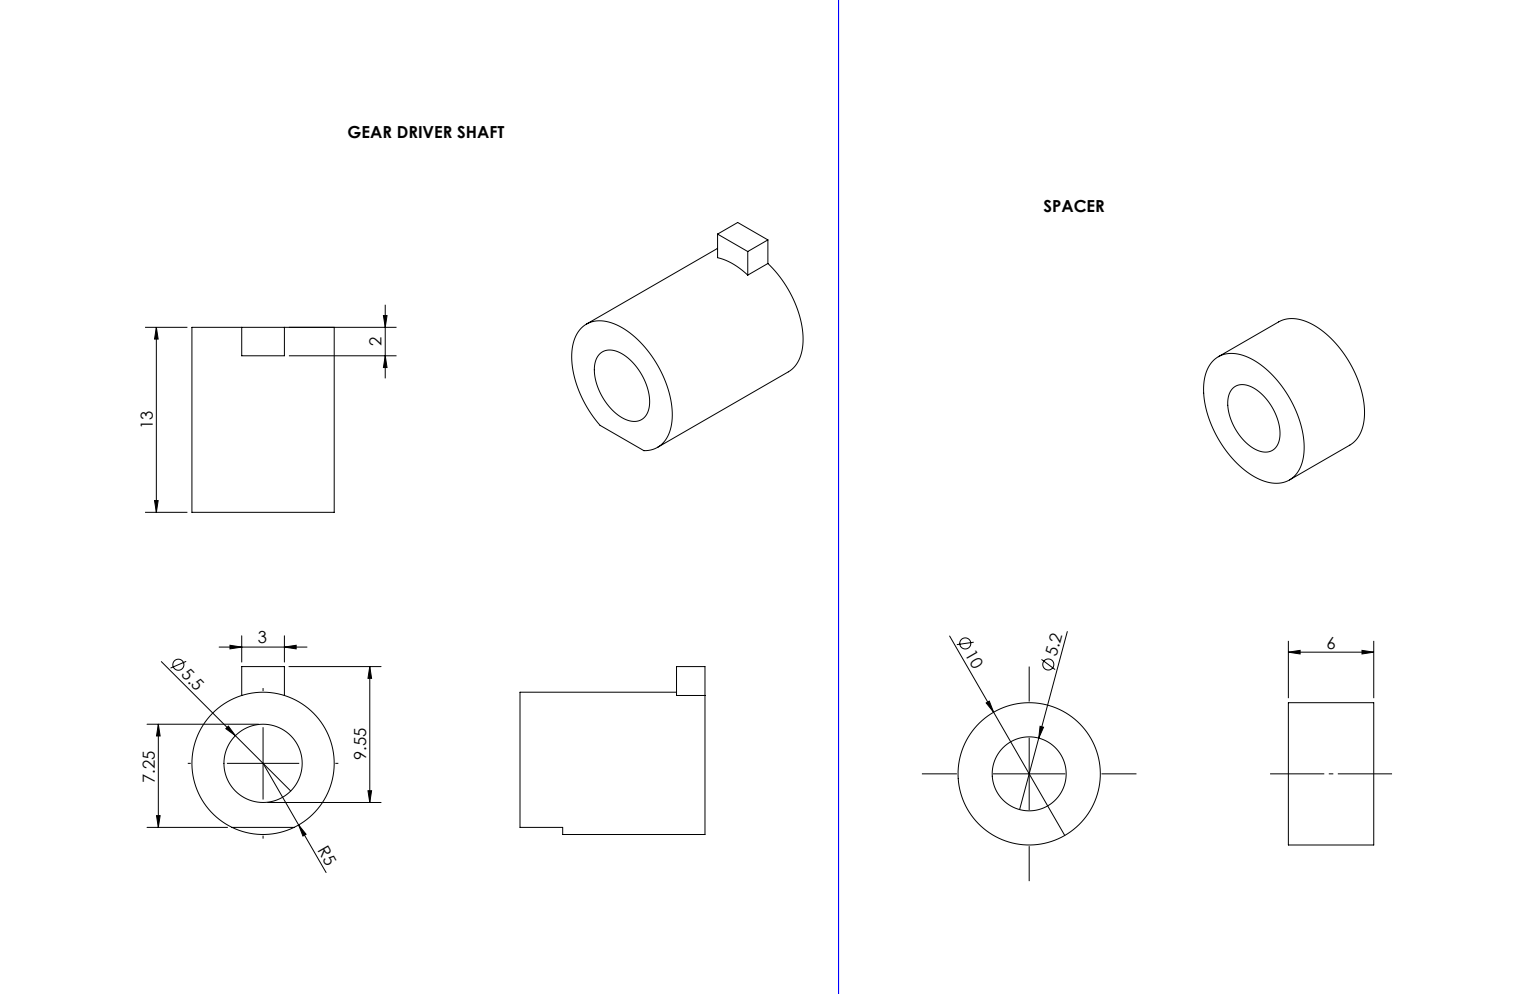
ISO-10303-21;
HEADER;
FILE_DESCRIPTION (('STEP AP214'),
    '1' );
FILE_NAME ('spacer.step',
    '2026-09-24T10:15:42',
    ( '' ),
    ( '' ),
    'SwSTEP 2.0',
    'SolidWorks 2026',
    '' );
FILE_SCHEMA (( 'AUTOMOTIVE_DESIGN' ));
ENDSEC;

DATA;
#16=( NAMED_UNIT ( * ) SI_UNIT ( $, .STERADIAN. ) SOLID_ANGLE_UNIT ( ) );
#41=UNCERTAINTY_MEASURE_WITH_UNIT (LENGTH_MEASURE( 1.000000000000000082E-05 ), #17046, 'distance_accuracy_value', 'NONE');
#42=PRODUCT_DEFINITION_SHAPE ( 'NONE', 'NONE',  #2847 ) ;
#65=CARTESIAN_POINT ( 'NONE',  ( -110.4113270445337918, -81.60345299795268659, -91.28051051278382033 ) ) ;
#145=AXIS2_PLACEMENT_3D ( 'NONE', #9237, #166, #12114 ) ;
#166=DIRECTION ( 'NONE',  ( -0.4246593920385851040, -0.1376957914266804250, 0.8948208031649687033 ) ) ;
#172=ADVANCED_FACE ( 'NONE', ( #1954 ), #15138, .T. ) ;
#207=UNCERTAINTY_MEASURE_WITH_UNIT (LENGTH_MEASURE( 1.000000000000000082E-05 ), #5383, 'distance_accuracy_value', 'NONE');
#238=CARTESIAN_POINT ( 'NONE',  ( -114.9284586926032574, -81.60345299795268659, -93.42422730238307338 ) ) ;
#331=ORIENTED_EDGE ( 'NONE', *, *, #11334, .T. ) ;
#403=EDGE_CURVE ( 'NONE', #15002, #6105, #16927, .T. ) ;
#642=CARTESIAN_POINT ( 'NONE',  ( -108.0624185875376639, -81.60345299795268659, -90.16577778219220818 ) ) ;
#654=ORIENTED_EDGE ( 'NONE', *, *, #12850, .T. ) ;
#822=DIRECTION ( 'NONE',  ( -0.4246593920385850485, -0.1376957914266803973, 0.8948208031649685923 ) ) ;
#900=SURFACE_STYLE_USAGE ( .BOTH. , #17132 ) ;
#954=ORIENTED_EDGE ( 'NONE', *, *, #11160, .F. ) ;
#1205=DIRECTION ( 'NONE',  ( -0.9034263296138843602, 0.000000000000000000, -0.4287433579198459133 ) ) ;
#1243=CIRCLE ( 'NONE', #11940, 2.600000000000039613 ) ;
#1307=EDGE_CURVE ( 'NONE', #11625, #16657, #17189, .T. ) ;
#1954=FACE_OUTER_BOUND ( 'NONE', #12857, .T. ) ;
#2030=AXIS2_PLACEMENT_3D ( 'NONE', #15716, #11248, #17249 ) ;
#2047=DIRECTION ( 'NONE',  ( -0.4246593920385851040, -0.1376957914266804250, 0.8948208031649687033 ) ) ;
#2160=CYLINDRICAL_SURFACE ( 'NONE', #10914, 2.600000000000039613 ) ;
#2164=ADVANCED_FACE ( 'NONE', ( #8660, #4276 ), #16018, .T. ) ;
#2283=AXIS2_PLACEMENT_3D ( 'NONE', #65, #14490, #17085 ) ;
#2304=ADVANCED_FACE ( 'NONE', ( #6184 ), #17755, .F. ) ;
#2329=( GEOMETRIC_REPRESENTATION_CONTEXT ( 3 ) GLOBAL_UNCERTAINTY_ASSIGNED_CONTEXT ( ( #207 ) ) GLOBAL_UNIT_ASSIGNED_CONTEXT ( ( #5383, #4140, #9959 ) ) REPRESENTATION_CONTEXT ( 'NONE', 'WORKASPACE' ) );
#2333=CARTESIAN_POINT ( 'NONE',  ( -117.4764150448347806, -82.42962774651277869, -88.05530248339326249 ) ) ;
#2416=SHAPE_REPRESENTATION_RELATIONSHIP ( 'NONE' , 'NONE' ,  #14858, #5341 ) ;
#2753=FACE_OUTER_BOUND ( 'NONE', #18659, .T. ) ;
#2762=EDGE_LOOP ( 'NONE', ( #16095, #331, #5318, #17520 ) ) ;
#2836=ORIENTED_EDGE ( 'NONE', *, *, #9238, .F. ) ;
#2847=PRODUCT_DEFINITION ( 'UNKNOWN', '', #12632, #13642 ) ;
#2872=DIRECTION ( 'NONE',  ( 0.4246593920385850485, 0.1376957914266804250, -0.8948208031649687033 ) ) ;
#2882=VERTEX_POINT ( 'NONE', #18469 ) ;
#2961=( LENGTH_UNIT ( ) NAMED_UNIT ( * ) SI_UNIT ( .MILLI., .METRE. ) );
#3026=LINE ( 'NONE', #17381, #6256 ) ;
#3231=MECHANICAL_DESIGN_GEOMETRIC_PRESENTATION_REPRESENTATION('',(#9367),#5997);
#3582=DIRECTION ( 'NONE',  ( -0.9034263296138832500, 0.000000000000000000, -0.4287433579198481337 ) ) ;
#3586=CIRCLE ( 'NONE', #14264, 5.000000000000049738 ) ;
#3646=( GEOMETRIC_REPRESENTATION_CONTEXT ( 3 ) GLOBAL_UNCERTAINTY_ASSIGNED_CONTEXT ( ( #4038 ) ) GLOBAL_UNIT_ASSIGNED_CONTEXT ( ( #2961, #13298, #16 ) ) REPRESENTATION_CONTEXT ( 'NONE', 'WORKASPACE' ) );
#3668=CARTESIAN_POINT ( 'NONE',  ( -110.4113270445337918, -81.60345299795268659, -91.28051051278382033 ) ) ;
#3708=MANIFOLD_SOLID_BREP ( 'Boss-Extrude1', #4810 ) ;
#3926=DIRECTION ( 'NONE',  ( -0.4246593920385851040, -0.1376957914266804250, 0.8948208031649687033 ) ) ;
#3928=CARTESIAN_POINT ( 'NONE',  ( -105.8941953964643261, -81.60345299795268659, -89.13679372318456728 ) ) ;
#4038=UNCERTAINTY_MEASURE_WITH_UNIT (LENGTH_MEASURE( 1.000000000000000082E-05 ), #2961, 'distance_accuracy_value', 'NONE');
#4042=( NAMED_UNIT ( * ) PLANE_ANGLE_UNIT ( ) SI_UNIT ( $, .RADIAN. ) );
#4140=( NAMED_UNIT ( * ) PLANE_ANGLE_UNIT ( ) SI_UNIT ( $, .RADIAN. ) );
#4245=ORIENTED_EDGE ( 'NONE', *, *, #7685, .T. ) ;
#4276=FACE_BOUND ( 'NONE', #5652, .T. ) ;
#4295=DIRECTION ( 'NONE',  ( -0.4246593920385850485, -0.1376957914266803973, 0.8948208031649685923 ) ) ;
#4693=DIRECTION ( 'NONE',  ( 0.4246593920385850485, 0.1376957914266804250, -0.8948208031649687033 ) ) ;
#4810=CLOSED_SHELL ( 'NONE', ( #15173, #18029, #2164, #10355, #172, #2304 ) ) ;
#5006=AXIS2_PLACEMENT_3D ( 'NONE', #14426, #5913, #11854 ) ;
#5008=DIRECTION ( 'NONE',  ( 0.4246593920385850485, 0.1376957914266804250, -0.8948208031649687033 ) ) ;
#5232=VECTOR ( 'NONE', #17908, 1000.000000000000114 ) ;
#5318=ORIENTED_EDGE ( 'NONE', *, *, #9306, .T. ) ;
#5341=ADVANCED_BREP_SHAPE_REPRESENTATION ( '', ( #3708, #2030 ), #2329 ) ;
#5352=EDGE_LOOP ( 'NONE', ( #654, #10815 ) ) ;
#5369=AXIS2_PLACEMENT_3D ( 'NONE', #9493, #11119, #7983 ) ;
#5383=( LENGTH_UNIT ( ) NAMED_UNIT ( * ) SI_UNIT ( .MILLI., .METRE. ) );
#5652=EDGE_LOOP ( 'NONE', ( #2836, #954 ) ) ;
#5816=FACE_BOUND ( 'NONE', #5352, .T. ) ;
#5913=DIRECTION ( 'NONE',  ( 0.4246593920385849930, 0.1376957914266804250, -0.8948208031649685923 ) ) ;
#5945=CIRCLE ( 'NONE', #17552, 2.600000000000039613 ) ;
#5997=( GEOMETRIC_REPRESENTATION_CONTEXT ( 3 ) GLOBAL_UNCERTAINTY_ASSIGNED_CONTEXT ( ( #41 ) ) GLOBAL_UNIT_ASSIGNED_CONTEXT ( ( #17046, #4042, #9689 ) ) REPRESENTATION_CONTEXT ( 'NONE', 'WORKASPACE' ) );
#6029=ORIENTED_EDGE ( 'NONE', *, *, #12850, .F. ) ;
#6076=APPLICATION_CONTEXT ( 'automotive_design' ) ;
#6105=VERTEX_POINT ( 'NONE', #7022 ) ;
#6179=ORIENTED_EDGE ( 'NONE', *, *, #9306, .F. ) ;
#6184=FACE_OUTER_BOUND ( 'NONE', #14679, .T. ) ;
#6206=CIRCLE ( 'NONE', #11097, 2.600000000000039613 ) ;
#6256=VECTOR ( 'NONE', #4295, 1000.000000000000114 ) ;
#6299=ORIENTED_EDGE ( 'NONE', *, *, #403, .F. ) ;
#6320=DIRECTION ( 'NONE',  ( -0.9034263296138832500, 0.000000000000000000, -0.4287433579198481337 ) ) ;
#6557=CARTESIAN_POINT ( 'NONE',  ( -110.4113270445337918, -81.60345299795268659, -91.28051051278382033 ) ) ;
#6644=CARTESIAN_POINT ( 'NONE',  ( -112.7602355015299338, -81.60345299795268659, -92.39524324337544670 ) ) ;
#6740=PRESENTATION_STYLE_ASSIGNMENT (( #900 ) ) ;
#6953=ORIENTED_EDGE ( 'NONE', *, *, #8829, .F. ) ;
#6958=ORIENTED_EDGE ( 'NONE', *, *, #11334, .F. ) ;
#7022=CARTESIAN_POINT ( 'NONE',  ( -110.6103749397691729, -82.42962774651277869, -84.79685296320238308 ) ) ;
#7095=SURFACE_SIDE_STYLE ('',( #16069 ) ) ;
#7685=EDGE_CURVE ( 'NONE', #11625, #15676, #3026, .T. ) ;
#7983=DIRECTION ( 'NONE',  ( -0.9034263296138832500, 0.000000000000000000, -0.4287433579198481337 ) ) ;
#8229=COLOUR_RGB ( '', 0.40784314, 0.44705882, 0.49803922) ;
#8353=LINE ( 'NONE', #12826, #8638 ) ;
#8463=CIRCLE ( 'NONE', #16717, 5.000000000000049738 ) ;
#8477=DIRECTION ( 'NONE',  ( 0.4246593920385850485, 0.1376957914266804250, -0.8948208031649687033 ) ) ;
#8526=FILL_AREA_STYLE ('',( #9952 ) ) ;
#8545=ORIENTED_EDGE ( 'NONE', *, *, #1307, .T. ) ;
#8601=PLANE ( 'NONE',  #5006 ) ;
#8638=VECTOR ( 'NONE', #14170, 1000.000000000000114 ) ;
#8660=FACE_OUTER_BOUND ( 'NONE', #13052, .T. ) ;
#8721=VECTOR ( 'NONE', #822, 1000.000000000000114 ) ;
#8823=EDGE_LOOP ( 'NONE', ( #11004, #12491, #6029, #6953 ) ) ;
#8829=EDGE_CURVE ( 'NONE', #2882, #6105, #18394, .T. ) ;
#8988=DIRECTION ( 'NONE',  ( 0.4246593920385850485, 0.1376957914266804250, -0.8948208031649687033 ) ) ;
#9233=VERTEX_POINT ( 'NONE', #6644 ) ;
#9237=CARTESIAN_POINT ( 'NONE',  ( -110.4113270445337918, -81.60345299795268659, -91.28051051278382033 ) ) ;
#9238=EDGE_CURVE ( 'NONE', #2882, #9233, #5945, .T. ) ;
#9306=EDGE_CURVE ( 'NONE', #14151, #15676, #11150, .T. ) ;
#9367=STYLED_ITEM ( 'NONE', ( #6740 ), #5341 ) ;
#9415=SHAPE_DEFINITION_REPRESENTATION ( #42, #14858 ) ;
#9493=CARTESIAN_POINT ( 'NONE',  ( -112.9592833967653149, -82.42962774651277869, -85.91158569379400944 ) ) ;
#9503=DIRECTION ( 'NONE',  ( 0.4246593920385850485, 0.1376957914266804250, -0.8948208031649687033 ) ) ;
#9689=( NAMED_UNIT ( * ) SI_UNIT ( $, .STERADIAN. ) SOLID_ANGLE_UNIT ( ) );
#9952=FILL_AREA_STYLE_COLOUR ( '', #8229 ) ;
#9959=( NAMED_UNIT ( * ) SI_UNIT ( $, .STERADIAN. ) SOLID_ANGLE_UNIT ( ) );
#10159=ORIENTED_EDGE ( 'NONE', *, *, #15741, .T. ) ;
#10224=AXIS2_PLACEMENT_3D ( 'NONE', #12546, #18377, #13712 ) ;
#10340=SURFACE_STYLE_USAGE ( .BOTH. , #7095 ) ;
#10354=ORIENTED_EDGE ( 'NONE', *, *, #1307, .F. ) ;
#10355=ADVANCED_FACE ( 'NONE', ( #2753, #5816 ), #8601, .F. ) ;
#10374=CARTESIAN_POINT ( 'NONE',  ( -115.3081918537614428, -82.42962774651277869, -87.02631842438563581 ) ) ;
#10815=ORIENTED_EDGE ( 'NONE', *, *, #403, .T. ) ;
#10855=PRODUCT_CONTEXT ( 'NONE', #6076, 'mechanical' ) ;
#10914=AXIS2_PLACEMENT_3D ( 'NONE', #6557, #12377, #15332 ) ;
#11004=ORIENTED_EDGE ( 'NONE', *, *, #9238, .T. ) ;
#11097=AXIS2_PLACEMENT_3D ( 'NONE', #12373, #9503, #3582 ) ;
#11119=DIRECTION ( 'NONE',  ( 0.4246593920385850485, 0.1376957914266804250, -0.8948208031649687033 ) ) ;
#11128=DIRECTION ( 'NONE',  ( -0.9034263296138832500, 0.000000000000000000, -0.4287433579198481337 ) ) ;
#11150=CIRCLE ( 'NONE', #10224, 5.000000000000049738 ) ;
#11160=EDGE_CURVE ( 'NONE', #9233, #2882, #6206, .T. ) ;
#11202=CARTESIAN_POINT ( 'NONE',  ( -110.4113270445337918, -81.60345299795268659, -91.28051051278382033 ) ) ;
#11248=DIRECTION ( 'NONE',  ( 0.000000000000000000, 0.000000000000000000, 1.000000000000000000 ) ) ;
#11334=EDGE_CURVE ( 'NONE', #16657, #14151, #8353, .T. ) ;
#11502=FILL_AREA_STYLE_COLOUR ( '', #14237 ) ;
#11625=VERTEX_POINT ( 'NONE', #3928 ) ;
#11854=DIRECTION ( 'NONE',  ( -0.9034263296138842492, 0.000000000000000000, -0.4287433579198461908 ) ) ;
#11862=CARTESIAN_POINT ( 'NONE',  ( -108.4421517486958351, -82.42962774651277869, -83.76786890419475640 ) ) ;
#11940=AXIS2_PLACEMENT_3D ( 'NONE', #17790, #4693, #6320 ) ;
#11962=PRODUCT ( 'spacer', 'spacer', '', ( #10855 ) ) ;
#12031=ORIENTED_EDGE ( 'NONE', *, *, #11160, .T. ) ;
#12067=AXIS2_PLACEMENT_3D ( 'NONE', #11202, #3926, #13617 ) ;
#12075=LINE ( 'NONE', #13781, #5232 ) ;
#12114=DIRECTION ( 'NONE',  ( 0.9034263296138832500, 0.000000000000000000, 0.4287433579198481337 ) ) ;
#12373=CARTESIAN_POINT ( 'NONE',  ( -110.4113270445337918, -81.60345299795268659, -91.28051051278382033 ) ) ;
#12377=DIRECTION ( 'NONE',  ( -0.4246593920385851040, -0.1376957914266804250, 0.8948208031649687033 ) ) ;
#12491=ORIENTED_EDGE ( 'NONE', *, *, #12587, .T. ) ;
#12546=CARTESIAN_POINT ( 'NONE',  ( -112.9592833967653149, -82.42962774651277869, -85.91158569379400944 ) ) ;
#12587=EDGE_CURVE ( 'NONE', #9233, #15002, #12075, .T. ) ;
#12632=PRODUCT_DEFINITION_FORMATION_WITH_SPECIFIED_SOURCE ( 'ANY', '', #11962, .NOT_KNOWN. ) ;
#12826=CARTESIAN_POINT ( 'NONE',  ( -114.9284586926032574, -81.60345299795268659, -93.42422730238307338 ) ) ;
#12850=EDGE_CURVE ( 'NONE', #6105, #15002, #1243, .T. ) ;
#12857=EDGE_LOOP ( 'NONE', ( #6958, #10354, #4245, #10159 ) ) ;
#13052=EDGE_LOOP ( 'NONE', ( #8545, #15213 ) ) ;
#13298=( NAMED_UNIT ( * ) PLANE_ANGLE_UNIT ( ) SI_UNIT ( $, .RADIAN. ) );
#13380=AXIS2_PLACEMENT_3D ( 'NONE', #14847, #2047, #17918 ) ;
#13416=MECHANICAL_DESIGN_GEOMETRIC_PRESENTATION_REPRESENTATION('',(#13725),#3646);
#13520=APPLICATION_CONTEXT ( 'automotive_design' ) ;
#13617=DIRECTION ( 'NONE',  ( 0.9034263296138843602, 0.000000000000000000, 0.4287433579198459133 ) ) ;
#13642=PRODUCT_DEFINITION_CONTEXT ( 'detailed design', #13520, 'design' ) ;
#13712=DIRECTION ( 'NONE',  ( -0.9034263296138843602, 0.000000000000000000, -0.4287433579198459133 ) ) ;
#13725=STYLED_ITEM ( 'NONE', ( #15785 ), #3708 ) ;
#13728=ORIENTED_EDGE ( 'NONE', *, *, #8829, .T. ) ;
#13781=CARTESIAN_POINT ( 'NONE',  ( -112.7602355015299338, -81.60345299795268659, -92.39524324337544670 ) ) ;
#14151=VERTEX_POINT ( 'NONE', #2333 ) ;
#14170=DIRECTION ( 'NONE',  ( -0.4246593920385850485, -0.1376957914266803973, 0.8948208031649685923 ) ) ;
#14237=COLOUR_RGB ( '', 0.40784314, 0.44705882, 0.49803922) ;
#14264=AXIS2_PLACEMENT_3D ( 'NONE', #17702, #8988, #14816 ) ;
#14426=CARTESIAN_POINT ( 'NONE',  ( -112.9592833967653149, -82.42962774651277869, -85.91158569379400944 ) ) ;
#14490=DIRECTION ( 'NONE',  ( 0.4246593920385849930, 0.1376957914266804250, -0.8948208031649685923 ) ) ;
#14551=DIRECTION ( 'NONE',  ( -0.9034263296138843602, 0.000000000000000000, -0.4287433579198459133 ) ) ;
#14679=EDGE_LOOP ( 'NONE', ( #18007, #12031, #13728, #6299 ) ) ;
#14816=DIRECTION ( 'NONE',  ( -0.9034263296138843602, 0.000000000000000000, -0.4287433579198459133 ) ) ;
#14847=CARTESIAN_POINT ( 'NONE',  ( -110.4113270445337918, -81.60345299795268659, -91.28051051278382033 ) ) ;
#14858=SHAPE_REPRESENTATION ( 'spacer', ( #2030 ), #2329 ) ;
#14951=FACE_OUTER_BOUND ( 'NONE', #2762, .T. ) ;
#15002=VERTEX_POINT ( 'NONE', #10374 ) ;
#15138=CYLINDRICAL_SURFACE ( 'NONE', #13380, 5.000000000000049738 ) ;
#15173=ADVANCED_FACE ( 'NONE', ( #16593 ), #2160, .F. ) ;
#15213=ORIENTED_EDGE ( 'NONE', *, *, #15403, .T. ) ;
#15332=DIRECTION ( 'NONE',  ( 0.9034263296138832500, 0.000000000000000000, 0.4287433579198481337 ) ) ;
#15403=EDGE_CURVE ( 'NONE', #16657, #11625, #8463, .T. ) ;
#15676=VERTEX_POINT ( 'NONE', #11862 ) ;
#15716=CARTESIAN_POINT ( 'NONE',  ( 0.000000000000000000, 0.000000000000000000, 0.000000000000000000 ) ) ;
#15728=CARTESIAN_POINT ( 'NONE',  ( -110.4113270445337918, -81.60345299795268659, -91.28051051278382033 ) ) ;
#15741=EDGE_CURVE ( 'NONE', #15676, #14151, #3586, .T. ) ;
#15785=PRESENTATION_STYLE_ASSIGNMENT (( #10340 ) ) ;
#16018=PLANE ( 'NONE',  #2283 ) ;
#16069=SURFACE_STYLE_FILL_AREA ( #8526 ) ;
#16095=ORIENTED_EDGE ( 'NONE', *, *, #15403, .F. ) ;
#16282=CARTESIAN_POINT ( 'NONE',  ( -110.4113270445337918, -81.60345299795268659, -91.28051051278382033 ) ) ;
#16529=ORIENTED_EDGE ( 'NONE', *, *, #15741, .F. ) ;
#16593=FACE_OUTER_BOUND ( 'NONE', #8823, .T. ) ;
#16657=VERTEX_POINT ( 'NONE', #238 ) ;
#16717=AXIS2_PLACEMENT_3D ( 'NONE', #16282, #2872, #14551 ) ;
#16927=CIRCLE ( 'NONE', #5369, 2.600000000000039613 ) ;
#16953=FILL_AREA_STYLE ('',( #11502 ) ) ;
#17046=( LENGTH_UNIT ( ) NAMED_UNIT ( * ) SI_UNIT ( .MILLI., .METRE. ) );
#17085=DIRECTION ( 'NONE',  ( -0.9034263296138842492, 0.000000000000000000, -0.4287433579198461908 ) ) ;
#17132=SURFACE_SIDE_STYLE ('',( #17320 ) ) ;
#17189=CIRCLE ( 'NONE', #18708, 5.000000000000049738 ) ;
#17249=DIRECTION ( 'NONE',  ( 1.000000000000000000, 0.000000000000000000, 0.000000000000000000 ) ) ;
#17320=SURFACE_STYLE_FILL_AREA ( #16953 ) ;
#17381=CARTESIAN_POINT ( 'NONE',  ( -105.8941953964643261, -81.60345299795268659, -89.13679372318456728 ) ) ;
#17520=ORIENTED_EDGE ( 'NONE', *, *, #7685, .F. ) ;
#17552=AXIS2_PLACEMENT_3D ( 'NONE', #3668, #5008, #11128 ) ;
#17702=CARTESIAN_POINT ( 'NONE',  ( -112.9592833967653149, -82.42962774651277869, -85.91158569379400944 ) ) ;
#17755=CYLINDRICAL_SURFACE ( 'NONE', #145, 2.600000000000039613 ) ;
#17790=CARTESIAN_POINT ( 'NONE',  ( -112.9592833967653149, -82.42962774651277869, -85.91158569379400944 ) ) ;
#17830=CYLINDRICAL_SURFACE ( 'NONE', #12067, 5.000000000000049738 ) ;
#17908=DIRECTION ( 'NONE',  ( -0.4246593920385850485, -0.1376957914266803973, 0.8948208031649685923 ) ) ;
#17918=DIRECTION ( 'NONE',  ( 0.9034263296138843602, 0.000000000000000000, 0.4287433579198459133 ) ) ;
#18007=ORIENTED_EDGE ( 'NONE', *, *, #12587, .F. ) ;
#18029=ADVANCED_FACE ( 'NONE', ( #14951 ), #17830, .T. ) ;
#18377=DIRECTION ( 'NONE',  ( 0.4246593920385850485, 0.1376957914266804250, -0.8948208031649687033 ) ) ;
#18394=LINE ( 'NONE', #642, #8721 ) ;
#18469=CARTESIAN_POINT ( 'NONE',  ( -108.0624185875376639, -81.60345299795268659, -90.16577778219220818 ) ) ;
#18659=EDGE_LOOP ( 'NONE', ( #16529, #6179 ) ) ;
#18708=AXIS2_PLACEMENT_3D ( 'NONE', #15728, #8477, #1205 ) ;
ENDSEC;
END-ISO-10303-21;
